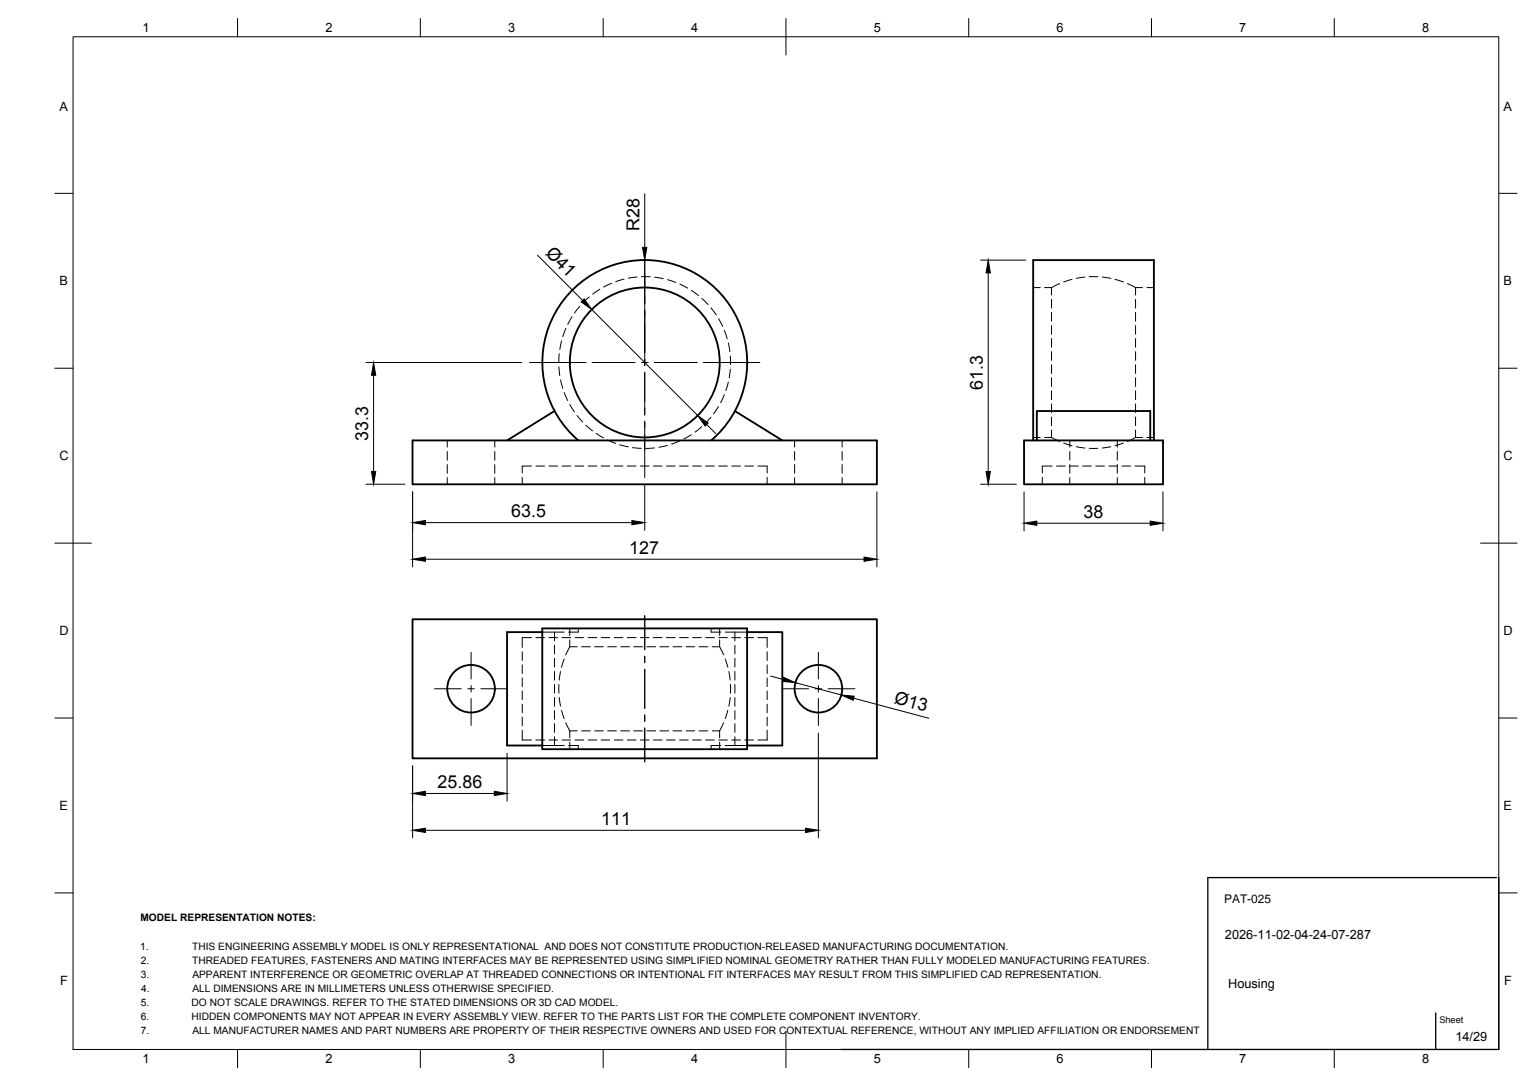
ISO-10303-21;
HEADER;
/* Generated by software containing ST-Developer
 * from STEP Tools, Inc. (www.steptools.com) 
 */

FILE_DESCRIPTION(
/* description */ ('Counter shaft with two pulleys and keyed hub'),
/* implementation_level */ '2;1');

FILE_NAME(
/* name */ 'Housing.step',
/* time_stamp */ '2026-10-27T10:46:10-07:00',
/* author */ (''),
/* organization */ (''),
/* preprocessor_version */ 'ST-DEVELOPER v20.2',
/* originating_system */ 'Autodesk Translation Framework v15.17.0.0',
/* authorisation */ '');

FILE_SCHEMA (('AUTOMOTIVE_DESIGN { 1 0 10303 214 3 1 1 }'));
ENDSEC;

DATA;
#10=MECHANICAL_DESIGN_GEOMETRIC_PRESENTATION_REPRESENTATION('',(#297),#10821);
#238=SPHERICAL_SURFACE('',#5956,2.35);
#247=SHAPE_REPRESENTATION_RELATIONSHIP('SRR','None',#10934,#272);
#272=ADVANCED_BREP_SHAPE_REPRESENTATION('',(#323),#10802);
#297=STYLED_ITEM('',(#11114),#323);
#323=MANIFOLD_SOLID_BREP('Body1',#5580);
#356=FACE_BOUND('',#959,.T.);
#357=FACE_BOUND('',#960,.T.);
#358=FACE_BOUND('',#968,.T.);
#359=FACE_BOUND('',#969,.T.);
#360=FACE_BOUND('',#970,.T.);
#361=FACE_BOUND('',#973,.T.);
#362=FACE_BOUND('',#975,.T.);
#363=FACE_BOUND('',#988,.T.);
#364=FACE_BOUND('',#989,.T.);
#365=FACE_BOUND('',#990,.T.);
#457=PLANE('',#5958);
#458=PLANE('',#5960);
#459=PLANE('',#5962);
#460=PLANE('',#5964);
#461=PLANE('',#5965);
#462=PLANE('',#5967);
#463=PLANE('',#5968);
#464=PLANE('',#5974);
#465=PLANE('',#5975);
#466=PLANE('',#5976);
#467=PLANE('',#5977);
#468=PLANE('',#5978);
#469=PLANE('',#5979);
#470=PLANE('',#5980);
#471=PLANE('',#5985);
#472=PLANE('',#5986);
#473=PLANE('',#5987);
#474=PLANE('',#5988);
#475=PLANE('',#5989);
#626=FACE_OUTER_BOUND('',#956,.T.);
#627=FACE_OUTER_BOUND('',#957,.T.);
#628=FACE_OUTER_BOUND('',#958,.T.);
#629=FACE_OUTER_BOUND('',#961,.T.);
#630=FACE_OUTER_BOUND('',#962,.T.);
#631=FACE_OUTER_BOUND('',#963,.T.);
#632=FACE_OUTER_BOUND('',#964,.T.);
#633=FACE_OUTER_BOUND('',#965,.T.);
#634=FACE_OUTER_BOUND('',#966,.T.);
#635=FACE_OUTER_BOUND('',#967,.T.);
#636=FACE_OUTER_BOUND('',#971,.T.);
#637=FACE_OUTER_BOUND('',#972,.T.);
#638=FACE_OUTER_BOUND('',#974,.T.);
#639=FACE_OUTER_BOUND('',#976,.T.);
#640=FACE_OUTER_BOUND('',#977,.T.);
#641=FACE_OUTER_BOUND('',#978,.T.);
#642=FACE_OUTER_BOUND('',#979,.T.);
#643=FACE_OUTER_BOUND('',#980,.T.);
#644=FACE_OUTER_BOUND('',#981,.T.);
#645=FACE_OUTER_BOUND('',#982,.T.);
#646=FACE_OUTER_BOUND('',#983,.T.);
#647=FACE_OUTER_BOUND('',#984,.T.);
#648=FACE_OUTER_BOUND('',#985,.T.);
#649=FACE_OUTER_BOUND('',#986,.T.);
#650=FACE_OUTER_BOUND('',#987,.T.);
#956=EDGE_LOOP('',(#3773,#3774,#3775,#3776));
#957=EDGE_LOOP('',(#3777,#3778,#3779,#3780));
#958=EDGE_LOOP('',(#3781,#3782));
#959=EDGE_LOOP('',(#3783));
#960=EDGE_LOOP('',(#3784));
#961=EDGE_LOOP('',(#3785,#3786,#3787));
#962=EDGE_LOOP('',(#3788,#3789,#3790));
#963=EDGE_LOOP('',(#3791,#3792,#3793));
#964=EDGE_LOOP('',(#3794,#3795,#3796,#3797));
#965=EDGE_LOOP('',(#3798,#3799,#3800));
#966=EDGE_LOOP('',(#3801,#3802,#3803,#3804));
#967=EDGE_LOOP('',(#3805,#3806,#3807,#3808));
#968=EDGE_LOOP('',(#3809));
#969=EDGE_LOOP('',(#3810));
#970=EDGE_LOOP('',(#3811,#3812,#3813,#3814,#3815,#3816,#3817,#3818,#3819,
#3820,#3821,#3822));
#971=EDGE_LOOP('',(#3823,#3824,#3825,#3826,#3827,#3828,#3829,#3830,#3831,
#3832,#3833,#3834));
#972=EDGE_LOOP('',(#3835,#3836));
#973=EDGE_LOOP('',(#3837));
#974=EDGE_LOOP('',(#3838,#3839));
#975=EDGE_LOOP('',(#3840));
#976=EDGE_LOOP('',(#3841,#3842,#3843,#3844));
#977=EDGE_LOOP('',(#3845,#3846,#3847,#3848));
#978=EDGE_LOOP('',(#3849,#3850,#3851,#3852));
#979=EDGE_LOOP('',(#3853,#3854,#3855,#3856));
#980=EDGE_LOOP('',(#3857,#3858,#3859,#3860));
#981=EDGE_LOOP('',(#3861,#3862,#3863,#3864));
#982=EDGE_LOOP('',(#3865,#3866,#3867,#3868));
#983=EDGE_LOOP('',(#3869,#3870,#3871,#3872));
#984=EDGE_LOOP('',(#3873,#3874,#3875,#3876));
#985=EDGE_LOOP('',(#3877,#3878,#3879,#3880));
#986=EDGE_LOOP('',(#3881,#3882,#3883,#3884));
#987=EDGE_LOOP('',(#3885,#3886,#3887,#3888));
#988=EDGE_LOOP('',(#3889,#3890,#3891,#3892));
#989=EDGE_LOOP('',(#3893));
#990=EDGE_LOOP('',(#3894));
#1355=LINE('',#8485,#1744);
#1356=LINE('',#8491,#1745);
#1357=LINE('',#8500,#1746);
#1358=LINE('',#8502,#1747);
#1359=LINE('',#8507,#1748);
#1360=LINE('',#8510,#1749);
#1361=LINE('',#8514,#1750);
#1362=LINE('',#8517,#1751);
#1363=LINE('',#8519,#1752);
#1364=LINE('',#8520,#1753);
#1365=LINE('',#8524,#1754);
#1366=LINE('',#8526,#1755);
#1367=LINE('',#8529,#1756);
#1368=LINE('',#8530,#1757);
#1369=LINE('',#8534,#1758);
#1370=LINE('',#8536,#1759);
#1371=LINE('',#8538,#1760);
#1372=LINE('',#8539,#1761);
#1373=LINE('',#8545,#1762);
#1374=LINE('',#8547,#1763);
#1375=LINE('',#8548,#1764);
#1376=LINE('',#8550,#1765);
#1377=LINE('',#8552,#1766);
#1378=LINE('',#8553,#1767);
#1379=LINE('',#8562,#1768);
#1380=LINE('',#8564,#1769);
#1381=LINE('',#8566,#1770);
#1382=LINE('',#8567,#1771);
#1383=LINE('',#8570,#1772);
#1384=LINE('',#8572,#1773);
#1385=LINE('',#8573,#1774);
#1386=LINE('',#8576,#1775);
#1387=LINE('',#8578,#1776);
#1388=LINE('',#8579,#1777);
#1389=LINE('',#8581,#1778);
#1390=LINE('',#8582,#1779);
#1391=LINE('',#8587,#1780);
#1392=LINE('',#8591,#1781);
#1393=LINE('',#8595,#1782);
#1394=LINE('',#8596,#1783);
#1395=LINE('',#8597,#1784);
#1396=LINE('',#8600,#1785);
#1397=LINE('',#8601,#1786);
#1398=LINE('',#8604,#1787);
#1399=LINE('',#8605,#1788);
#1400=LINE('',#8607,#1789);
#1744=VECTOR('',#6757,2.05);
#1745=VECTOR('',#6764,2.05);
#1746=VECTOR('',#6773,1.);
#1747=VECTOR('',#6774,1.);
#1748=VECTOR('',#6779,1.);
#1749=VECTOR('',#6782,1.);
#1750=VECTOR('',#6785,1.);
#1751=VECTOR('',#6788,1.);
#1752=VECTOR('',#6791,1.);
#1753=VECTOR('',#6792,1.);
#1754=VECTOR('',#6795,1.);
#1755=VECTOR('',#6796,1.);
#1756=VECTOR('',#6801,1.);
#1757=VECTOR('',#6802,1.);
#1758=VECTOR('',#6805,1.);
#1759=VECTOR('',#6806,1.);
#1760=VECTOR('',#6807,1.);
#1761=VECTOR('',#6808,1.);
#1762=VECTOR('',#6813,1.);
#1763=VECTOR('',#6814,1.);
#1764=VECTOR('',#6815,1.);
#1765=VECTOR('',#6816,1.);
#1766=VECTOR('',#6817,1.);
#1767=VECTOR('',#6818,1.);
#1768=VECTOR('',#6831,1.);
#1769=VECTOR('',#6832,1.);
#1770=VECTOR('',#6833,1.);
#1771=VECTOR('',#6834,1.);
#1772=VECTOR('',#6837,1.);
#1773=VECTOR('',#6838,1.);
#1774=VECTOR('',#6839,1.);
#1775=VECTOR('',#6842,1.);
#1776=VECTOR('',#6843,1.);
#1777=VECTOR('',#6844,1.);
#1778=VECTOR('',#6847,1.);
#1779=VECTOR('',#6848,1.);
#1780=VECTOR('',#6855,0.65);
#1781=VECTOR('',#6860,0.65);
#1782=VECTOR('',#6863,1.);
#1783=VECTOR('',#6864,1.);
#1784=VECTOR('',#6865,1.);
#1785=VECTOR('',#6868,1.);
#1786=VECTOR('',#6869,1.);
#1787=VECTOR('',#6872,1.);
#1788=VECTOR('',#6873,1.);
#1789=VECTOR('',#6876,1.);
#2109=CIRCLE('',#5951,2.05);
#2110=CIRCLE('',#5952,2.05);
#2111=CIRCLE('',#5954,2.05);
#2112=CIRCLE('',#5955,2.05);
#2113=CIRCLE('',#5957,2.35);
#2114=CIRCLE('',#5959,2.8);
#2115=CIRCLE('',#5961,2.8);
#2116=CIRCLE('',#5963,2.8);
#2117=CIRCLE('',#5966,2.8);
#2118=CIRCLE('',#5969,0.65);
#2119=CIRCLE('',#5970,0.65);
#2120=CIRCLE('',#5972,2.8);
#2121=CIRCLE('',#5973,2.8);
#2122=CIRCLE('',#5982,0.65);
#2123=CIRCLE('',#5984,0.65);
#2432=VERTEX_POINT('',#8482);
#2433=VERTEX_POINT('',#8484);
#2434=VERTEX_POINT('',#8488);
#2435=VERTEX_POINT('',#8490);
#2436=VERTEX_POINT('',#8494);
#2437=VERTEX_POINT('',#8495);
#2438=VERTEX_POINT('',#8498);
#2439=VERTEX_POINT('',#8499);
#2440=VERTEX_POINT('',#8501);
#2441=VERTEX_POINT('',#8505);
#2442=VERTEX_POINT('',#8506);
#2443=VERTEX_POINT('',#8508);
#2444=VERTEX_POINT('',#8512);
#2445=VERTEX_POINT('',#8513);
#2446=VERTEX_POINT('',#8515);
#2447=VERTEX_POINT('',#8522);
#2448=VERTEX_POINT('',#8523);
#2449=VERTEX_POINT('',#8525);
#2450=VERTEX_POINT('',#8532);
#2451=VERTEX_POINT('',#8533);
#2452=VERTEX_POINT('',#8535);
#2453=VERTEX_POINT('',#8537);
#2454=VERTEX_POINT('',#8540);
#2455=VERTEX_POINT('',#8542);
#2456=VERTEX_POINT('',#8544);
#2457=VERTEX_POINT('',#8546);
#2458=VERTEX_POINT('',#8549);
#2459=VERTEX_POINT('',#8551);
#2460=VERTEX_POINT('',#8560);
#2461=VERTEX_POINT('',#8561);
#2462=VERTEX_POINT('',#8563);
#2463=VERTEX_POINT('',#8565);
#2464=VERTEX_POINT('',#8569);
#2465=VERTEX_POINT('',#8571);
#2466=VERTEX_POINT('',#8575);
#2467=VERTEX_POINT('',#8577);
#2468=VERTEX_POINT('',#8585);
#2469=VERTEX_POINT('',#8589);
#2470=VERTEX_POINT('',#8593);
#2471=VERTEX_POINT('',#8594);
#2472=VERTEX_POINT('',#8599);
#2473=VERTEX_POINT('',#8603);
#2959=EDGE_CURVE('',#2432,#2432,#2109,.T.);
#2960=EDGE_CURVE('',#2432,#2433,#1355,.T.);
#2961=EDGE_CURVE('',#2433,#2433,#2110,.T.);
#2962=EDGE_CURVE('',#2434,#2434,#2111,.T.);
#2963=EDGE_CURVE('',#2434,#2435,#1356,.T.);
#2964=EDGE_CURVE('',#2435,#2435,#2112,.T.);
#2965=EDGE_CURVE('',#2436,#2437,#2113,.T.);
#2966=EDGE_CURVE('',#2438,#2439,#1357,.T.);
#2967=EDGE_CURVE('',#2438,#2440,#1358,.T.);
#2968=EDGE_CURVE('',#2439,#2440,#2114,.T.);
#2969=EDGE_CURVE('',#2441,#2442,#1359,.T.);
#2970=EDGE_CURVE('',#2443,#2441,#2115,.T.);
#2971=EDGE_CURVE('',#2443,#2442,#1360,.T.);
#2972=EDGE_CURVE('',#2444,#2445,#1361,.T.);
#2973=EDGE_CURVE('',#2446,#2444,#2116,.T.);
#2974=EDGE_CURVE('',#2446,#2445,#1362,.T.);
#2975=EDGE_CURVE('',#2445,#2438,#1363,.T.);
#2976=EDGE_CURVE('',#2440,#2446,#1364,.T.);
#2977=EDGE_CURVE('',#2447,#2448,#1365,.T.);
#2978=EDGE_CURVE('',#2447,#2449,#1366,.T.);
#2979=EDGE_CURVE('',#2448,#2449,#2117,.T.);
#2980=EDGE_CURVE('',#2442,#2447,#1367,.T.);
#2981=EDGE_CURVE('',#2449,#2443,#1368,.T.);
#2982=EDGE_CURVE('',#2450,#2451,#1369,.T.);
#2983=EDGE_CURVE('',#2451,#2452,#1370,.T.);
#2984=EDGE_CURVE('',#2452,#2453,#1371,.T.);
#2985=EDGE_CURVE('',#2453,#2450,#1372,.T.);
#2986=EDGE_CURVE('',#2454,#2454,#2118,.T.);
#2987=EDGE_CURVE('',#2455,#2455,#2119,.T.);
#2988=EDGE_CURVE('',#2448,#2456,#1373,.T.);
#2989=EDGE_CURVE('',#2456,#2457,#1374,.T.);
#2990=EDGE_CURVE('',#2457,#2444,#1375,.T.);
#2991=EDGE_CURVE('',#2439,#2458,#1376,.T.);
#2992=EDGE_CURVE('',#2458,#2459,#1377,.T.);
#2993=EDGE_CURVE('',#2459,#2441,#1378,.T.);
#2994=EDGE_CURVE('',#2458,#2459,#2120,.T.);
#2995=EDGE_CURVE('',#2456,#2457,#2121,.T.);
#2996=EDGE_CURVE('',#2460,#2461,#1379,.T.);
#2997=EDGE_CURVE('',#2460,#2462,#1380,.T.);
#2998=EDGE_CURVE('',#2462,#2463,#1381,.T.);
#2999=EDGE_CURVE('',#2461,#2463,#1382,.T.);
#3000=EDGE_CURVE('',#2464,#2460,#1383,.T.);
#3001=EDGE_CURVE('',#2464,#2465,#1384,.T.);
#3002=EDGE_CURVE('',#2465,#2462,#1385,.T.);
#3003=EDGE_CURVE('',#2466,#2464,#1386,.T.);
#3004=EDGE_CURVE('',#2466,#2467,#1387,.T.);
#3005=EDGE_CURVE('',#2467,#2465,#1388,.T.);
#3006=EDGE_CURVE('',#2461,#2466,#1389,.T.);
#3007=EDGE_CURVE('',#2463,#2467,#1390,.T.);
#3008=EDGE_CURVE('',#2468,#2468,#2122,.T.);
#3009=EDGE_CURVE('',#2468,#2455,#1391,.T.);
#3010=EDGE_CURVE('',#2469,#2469,#2123,.T.);
#3011=EDGE_CURVE('',#2469,#2454,#1392,.T.);
#3012=EDGE_CURVE('',#2470,#2471,#1393,.T.);
#3013=EDGE_CURVE('',#2471,#2450,#1394,.T.);
#3014=EDGE_CURVE('',#2470,#2453,#1395,.T.);
#3015=EDGE_CURVE('',#2472,#2470,#1396,.T.);
#3016=EDGE_CURVE('',#2472,#2452,#1397,.T.);
#3017=EDGE_CURVE('',#2473,#2472,#1398,.T.);
#3018=EDGE_CURVE('',#2473,#2451,#1399,.T.);
#3019=EDGE_CURVE('',#2471,#2473,#1400,.T.);
#3773=ORIENTED_EDGE('',*,*,#2959,.F.);
#3774=ORIENTED_EDGE('',*,*,#2960,.T.);
#3775=ORIENTED_EDGE('',*,*,#2961,.F.);
#3776=ORIENTED_EDGE('',*,*,#2960,.F.);
#3777=ORIENTED_EDGE('',*,*,#2962,.F.);
#3778=ORIENTED_EDGE('',*,*,#2963,.T.);
#3779=ORIENTED_EDGE('',*,*,#2964,.F.);
#3780=ORIENTED_EDGE('',*,*,#2963,.F.);
#3781=ORIENTED_EDGE('',*,*,#2965,.T.);
#3782=ORIENTED_EDGE('',*,*,#2965,.F.);
#3783=ORIENTED_EDGE('',*,*,#2962,.T.);
#3784=ORIENTED_EDGE('',*,*,#2961,.T.);
#3785=ORIENTED_EDGE('',*,*,#2966,.F.);
#3786=ORIENTED_EDGE('',*,*,#2967,.T.);
#3787=ORIENTED_EDGE('',*,*,#2968,.F.);
#3788=ORIENTED_EDGE('',*,*,#2969,.F.);
#3789=ORIENTED_EDGE('',*,*,#2970,.F.);
#3790=ORIENTED_EDGE('',*,*,#2971,.T.);
#3791=ORIENTED_EDGE('',*,*,#2972,.F.);
#3792=ORIENTED_EDGE('',*,*,#2973,.F.);
#3793=ORIENTED_EDGE('',*,*,#2974,.T.);
#3794=ORIENTED_EDGE('',*,*,#2975,.F.);
#3795=ORIENTED_EDGE('',*,*,#2974,.F.);
#3796=ORIENTED_EDGE('',*,*,#2976,.F.);
#3797=ORIENTED_EDGE('',*,*,#2967,.F.);
#3798=ORIENTED_EDGE('',*,*,#2977,.F.);
#3799=ORIENTED_EDGE('',*,*,#2978,.T.);
#3800=ORIENTED_EDGE('',*,*,#2979,.F.);
#3801=ORIENTED_EDGE('',*,*,#2980,.F.);
#3802=ORIENTED_EDGE('',*,*,#2971,.F.);
#3803=ORIENTED_EDGE('',*,*,#2981,.F.);
#3804=ORIENTED_EDGE('',*,*,#2978,.F.);
#3805=ORIENTED_EDGE('',*,*,#2982,.T.);
#3806=ORIENTED_EDGE('',*,*,#2983,.T.);
#3807=ORIENTED_EDGE('',*,*,#2984,.T.);
#3808=ORIENTED_EDGE('',*,*,#2985,.T.);
#3809=ORIENTED_EDGE('',*,*,#2986,.T.);
#3810=ORIENTED_EDGE('',*,*,#2987,.T.);
#3811=ORIENTED_EDGE('',*,*,#2969,.T.);
#3812=ORIENTED_EDGE('',*,*,#2980,.T.);
#3813=ORIENTED_EDGE('',*,*,#2977,.T.);
#3814=ORIENTED_EDGE('',*,*,#2988,.T.);
#3815=ORIENTED_EDGE('',*,*,#2989,.T.);
#3816=ORIENTED_EDGE('',*,*,#2990,.T.);
#3817=ORIENTED_EDGE('',*,*,#2972,.T.);
#3818=ORIENTED_EDGE('',*,*,#2975,.T.);
#3819=ORIENTED_EDGE('',*,*,#2966,.T.);
#3820=ORIENTED_EDGE('',*,*,#2991,.T.);
#3821=ORIENTED_EDGE('',*,*,#2992,.T.);
#3822=ORIENTED_EDGE('',*,*,#2993,.T.);
#3823=ORIENTED_EDGE('',*,*,#2970,.T.);
#3824=ORIENTED_EDGE('',*,*,#2993,.F.);
#3825=ORIENTED_EDGE('',*,*,#2994,.F.);
#3826=ORIENTED_EDGE('',*,*,#2991,.F.);
#3827=ORIENTED_EDGE('',*,*,#2968,.T.);
#3828=ORIENTED_EDGE('',*,*,#2976,.T.);
#3829=ORIENTED_EDGE('',*,*,#2973,.T.);
#3830=ORIENTED_EDGE('',*,*,#2990,.F.);
#3831=ORIENTED_EDGE('',*,*,#2995,.F.);
#3832=ORIENTED_EDGE('',*,*,#2988,.F.);
#3833=ORIENTED_EDGE('',*,*,#2979,.T.);
#3834=ORIENTED_EDGE('',*,*,#2981,.T.);
#3835=ORIENTED_EDGE('',*,*,#2989,.F.);
#3836=ORIENTED_EDGE('',*,*,#2995,.T.);
#3837=ORIENTED_EDGE('',*,*,#2959,.T.);
#3838=ORIENTED_EDGE('',*,*,#2992,.F.);
#3839=ORIENTED_EDGE('',*,*,#2994,.T.);
#3840=ORIENTED_EDGE('',*,*,#2964,.T.);
#3841=ORIENTED_EDGE('',*,*,#2996,.F.);
#3842=ORIENTED_EDGE('',*,*,#2997,.T.);
#3843=ORIENTED_EDGE('',*,*,#2998,.T.);
#3844=ORIENTED_EDGE('',*,*,#2999,.F.);
#3845=ORIENTED_EDGE('',*,*,#3000,.F.);
#3846=ORIENTED_EDGE('',*,*,#3001,.T.);
#3847=ORIENTED_EDGE('',*,*,#3002,.T.);
#3848=ORIENTED_EDGE('',*,*,#2997,.F.);
#3849=ORIENTED_EDGE('',*,*,#3003,.F.);
#3850=ORIENTED_EDGE('',*,*,#3004,.T.);
#3851=ORIENTED_EDGE('',*,*,#3005,.T.);
#3852=ORIENTED_EDGE('',*,*,#3001,.F.);
#3853=ORIENTED_EDGE('',*,*,#3006,.F.);
#3854=ORIENTED_EDGE('',*,*,#2999,.T.);
#3855=ORIENTED_EDGE('',*,*,#3007,.T.);
#3856=ORIENTED_EDGE('',*,*,#3004,.F.);
#3857=ORIENTED_EDGE('',*,*,#3007,.F.);
#3858=ORIENTED_EDGE('',*,*,#2998,.F.);
#3859=ORIENTED_EDGE('',*,*,#3002,.F.);
#3860=ORIENTED_EDGE('',*,*,#3005,.F.);
#3861=ORIENTED_EDGE('',*,*,#3008,.F.);
#3862=ORIENTED_EDGE('',*,*,#3009,.T.);
#3863=ORIENTED_EDGE('',*,*,#2987,.F.);
#3864=ORIENTED_EDGE('',*,*,#3009,.F.);
#3865=ORIENTED_EDGE('',*,*,#3010,.F.);
#3866=ORIENTED_EDGE('',*,*,#3011,.T.);
#3867=ORIENTED_EDGE('',*,*,#2986,.F.);
#3868=ORIENTED_EDGE('',*,*,#3011,.F.);
#3869=ORIENTED_EDGE('',*,*,#3012,.T.);
#3870=ORIENTED_EDGE('',*,*,#3013,.T.);
#3871=ORIENTED_EDGE('',*,*,#2985,.F.);
#3872=ORIENTED_EDGE('',*,*,#3014,.F.);
#3873=ORIENTED_EDGE('',*,*,#3015,.T.);
#3874=ORIENTED_EDGE('',*,*,#3014,.T.);
#3875=ORIENTED_EDGE('',*,*,#2984,.F.);
#3876=ORIENTED_EDGE('',*,*,#3016,.F.);
#3877=ORIENTED_EDGE('',*,*,#3017,.T.);
#3878=ORIENTED_EDGE('',*,*,#3016,.T.);
#3879=ORIENTED_EDGE('',*,*,#2983,.F.);
#3880=ORIENTED_EDGE('',*,*,#3018,.F.);
#3881=ORIENTED_EDGE('',*,*,#3019,.T.);
#3882=ORIENTED_EDGE('',*,*,#3018,.T.);
#3883=ORIENTED_EDGE('',*,*,#2982,.F.);
#3884=ORIENTED_EDGE('',*,*,#3013,.F.);
#3885=ORIENTED_EDGE('',*,*,#3019,.F.);
#3886=ORIENTED_EDGE('',*,*,#3012,.F.);
#3887=ORIENTED_EDGE('',*,*,#3015,.F.);
#3888=ORIENTED_EDGE('',*,*,#3017,.F.);
#3889=ORIENTED_EDGE('',*,*,#2996,.T.);
#3890=ORIENTED_EDGE('',*,*,#3006,.T.);
#3891=ORIENTED_EDGE('',*,*,#3003,.T.);
#3892=ORIENTED_EDGE('',*,*,#3000,.T.);
#3893=ORIENTED_EDGE('',*,*,#3008,.T.);
#3894=ORIENTED_EDGE('',*,*,#3010,.T.);
#5125=CYLINDRICAL_SURFACE('',#5950,2.05);
#5126=CYLINDRICAL_SURFACE('',#5953,2.05);
#5127=CYLINDRICAL_SURFACE('',#5971,2.8);
#5128=CYLINDRICAL_SURFACE('',#5981,0.65);
#5129=CYLINDRICAL_SURFACE('',#5983,0.65);
#5297=ADVANCED_FACE('',(#626),#5125,.F.);
#5298=ADVANCED_FACE('',(#627),#5126,.F.);
#5299=ADVANCED_FACE('',(#628,#356,#357),#238,.F.);
#5300=ADVANCED_FACE('',(#629),#457,.T.);
#5301=ADVANCED_FACE('',(#630),#458,.T.);
#5302=ADVANCED_FACE('',(#631),#459,.T.);
#5303=ADVANCED_FACE('',(#632),#460,.T.);
#5304=ADVANCED_FACE('',(#633),#461,.T.);
#5305=ADVANCED_FACE('',(#634),#462,.T.);
#5306=ADVANCED_FACE('',(#635,#358,#359,#360),#463,.T.);
#5307=ADVANCED_FACE('',(#636),#5127,.T.);
#5308=ADVANCED_FACE('',(#637,#361),#464,.F.);
#5309=ADVANCED_FACE('',(#638,#362),#465,.T.);
#5310=ADVANCED_FACE('',(#639),#466,.F.);
#5311=ADVANCED_FACE('',(#640),#467,.F.);
#5312=ADVANCED_FACE('',(#641),#468,.F.);
#5313=ADVANCED_FACE('',(#642),#469,.F.);
#5314=ADVANCED_FACE('',(#643),#470,.F.);
#5315=ADVANCED_FACE('',(#644),#5128,.F.);
#5316=ADVANCED_FACE('',(#645),#5129,.F.);
#5317=ADVANCED_FACE('',(#646),#471,.T.);
#5318=ADVANCED_FACE('',(#647),#472,.T.);
#5319=ADVANCED_FACE('',(#648),#473,.T.);
#5320=ADVANCED_FACE('',(#649),#474,.T.);
#5321=ADVANCED_FACE('',(#650,#363,#364,#365),#475,.F.);
#5580=CLOSED_SHELL('',(#5297,#5298,#5299,#5300,#5301,#5302,#5303,#5304,
#5305,#5306,#5307,#5308,#5309,#5310,#5311,#5312,#5313,#5314,#5315,#5316,
#5317,#5318,#5319,#5320,#5321));
#5949=AXIS2_PLACEMENT_3D('',#8480,#6751,#6752);
#5950=AXIS2_PLACEMENT_3D('',#8481,#6753,#6754);
#5951=AXIS2_PLACEMENT_3D('',#8483,#6755,#6756);
#5952=AXIS2_PLACEMENT_3D('',#8486,#6758,#6759);
#5953=AXIS2_PLACEMENT_3D('',#8487,#6760,#6761);
#5954=AXIS2_PLACEMENT_3D('',#8489,#6762,#6763);
#5955=AXIS2_PLACEMENT_3D('',#8492,#6765,#6766);
#5956=AXIS2_PLACEMENT_3D('',#8493,#6767,#6768);
#5957=AXIS2_PLACEMENT_3D('',#8496,#6769,#6770);
#5958=AXIS2_PLACEMENT_3D('',#8497,#6771,#6772);
#5959=AXIS2_PLACEMENT_3D('',#8503,#6775,#6776);
#5960=AXIS2_PLACEMENT_3D('',#8504,#6777,#6778);
#5961=AXIS2_PLACEMENT_3D('',#8509,#6780,#6781);
#5962=AXIS2_PLACEMENT_3D('',#8511,#6783,#6784);
#5963=AXIS2_PLACEMENT_3D('',#8516,#6786,#6787);
#5964=AXIS2_PLACEMENT_3D('',#8518,#6789,#6790);
#5965=AXIS2_PLACEMENT_3D('',#8521,#6793,#6794);
#5966=AXIS2_PLACEMENT_3D('',#8527,#6797,#6798);
#5967=AXIS2_PLACEMENT_3D('',#8528,#6799,#6800);
#5968=AXIS2_PLACEMENT_3D('',#8531,#6803,#6804);
#5969=AXIS2_PLACEMENT_3D('',#8541,#6809,#6810);
#5970=AXIS2_PLACEMENT_3D('',#8543,#6811,#6812);
#5971=AXIS2_PLACEMENT_3D('',#8554,#6819,#6820);
#5972=AXIS2_PLACEMENT_3D('',#8555,#6821,#6822);
#5973=AXIS2_PLACEMENT_3D('',#8556,#6823,#6824);
#5974=AXIS2_PLACEMENT_3D('',#8557,#6825,#6826);
#5975=AXIS2_PLACEMENT_3D('',#8558,#6827,#6828);
#5976=AXIS2_PLACEMENT_3D('',#8559,#6829,#6830);
#5977=AXIS2_PLACEMENT_3D('',#8568,#6835,#6836);
#5978=AXIS2_PLACEMENT_3D('',#8574,#6840,#6841);
#5979=AXIS2_PLACEMENT_3D('',#8580,#6845,#6846);
#5980=AXIS2_PLACEMENT_3D('',#8583,#6849,#6850);
#5981=AXIS2_PLACEMENT_3D('',#8584,#6851,#6852);
#5982=AXIS2_PLACEMENT_3D('',#8586,#6853,#6854);
#5983=AXIS2_PLACEMENT_3D('',#8588,#6856,#6857);
#5984=AXIS2_PLACEMENT_3D('',#8590,#6858,#6859);
#5985=AXIS2_PLACEMENT_3D('',#8592,#6861,#6862);
#5986=AXIS2_PLACEMENT_3D('',#8598,#6866,#6867);
#5987=AXIS2_PLACEMENT_3D('',#8602,#6870,#6871);
#5988=AXIS2_PLACEMENT_3D('',#8606,#6874,#6875);
#5989=AXIS2_PLACEMENT_3D('',#8608,#6877,#6878);
#6751=DIRECTION('axis',(0.,0.,1.));
#6752=DIRECTION('refdir',(1.,0.,0.));
#6753=DIRECTION('center_axis',(0.,1.,0.));
#6754=DIRECTION('ref_axis',(1.,0.,0.));
#6755=DIRECTION('center_axis',(0.,1.,0.));
#6756=DIRECTION('ref_axis',(1.,0.,0.));
#6757=DIRECTION('',(0.,1.,0.));
#6758=DIRECTION('center_axis',(0.,-1.,0.));
#6759=DIRECTION('ref_axis',(1.,0.,0.));
#6760=DIRECTION('center_axis',(0.,1.,0.));
#6761=DIRECTION('ref_axis',(1.,0.,0.));
#6762=DIRECTION('center_axis',(0.,1.,0.));
#6763=DIRECTION('ref_axis',(1.,0.,0.));
#6764=DIRECTION('',(0.,1.,0.));
#6765=DIRECTION('center_axis',(0.,-1.,0.));
#6766=DIRECTION('ref_axis',(1.,0.,0.));
#6767=DIRECTION('center_axis',(6.12323399573677E-17,0.,1.));
#6768=DIRECTION('ref_axis',(1.,0.,0.));
#6769=DIRECTION('center_axis',(-1.22464679914735E-16,1.,0.));
#6770=DIRECTION('ref_axis',(-1.,-1.22464679914735E-16,0.));
#6771=DIRECTION('center_axis',(0.,1.,0.));
#6772=DIRECTION('ref_axis',(0.,0.,1.));
#6773=DIRECTION('',(1.,0.,0.));
#6774=DIRECTION('',(0.850265146687862,0.,0.526354614616295));
#6775=DIRECTION('center_axis',(0.,1.,0.));
#6776=DIRECTION('ref_axis',(1.,0.,0.));
#6777=DIRECTION('center_axis',(0.,1.,0.));
#6778=DIRECTION('ref_axis',(0.,0.,1.));
#6779=DIRECTION('',(1.,0.,0.));
#6780=DIRECTION('center_axis',(0.,1.,0.));
#6781=DIRECTION('ref_axis',(1.,0.,0.));
#6782=DIRECTION('',(0.850265146687862,0.,-0.526354614616295));
#6783=DIRECTION('center_axis',(0.,-1.,0.));
#6784=DIRECTION('ref_axis',(0.,0.,-1.));
#6785=DIRECTION('',(-1.,0.,0.));
#6786=DIRECTION('center_axis',(0.,-1.,0.));
#6787=DIRECTION('ref_axis',(1.,0.,0.));
#6788=DIRECTION('',(-0.850265146687862,0.,-0.526354614616295));
#6789=DIRECTION('center_axis',(-0.526354614616295,0.,0.850265146687862));
#6790=DIRECTION('ref_axis',(0.850265146687862,0.,0.526354614616295));
#6791=DIRECTION('',(0.,1.,0.));
#6792=DIRECTION('',(0.,-1.,0.));
#6793=DIRECTION('center_axis',(0.,-1.,0.));
#6794=DIRECTION('ref_axis',(0.,0.,-1.));
#6795=DIRECTION('',(-1.,0.,0.));
#6796=DIRECTION('',(-0.850265146687862,0.,0.526354614616295));
#6797=DIRECTION('center_axis',(0.,-1.,0.));
#6798=DIRECTION('ref_axis',(1.,0.,0.));
#6799=DIRECTION('center_axis',(0.526354614616295,0.,0.850265146687862));
#6800=DIRECTION('ref_axis',(0.850265146687862,0.,-0.526354614616295));
#6801=DIRECTION('',(0.,-1.,0.));
#6802=DIRECTION('',(0.,1.,0.));
#6803=DIRECTION('center_axis',(0.,0.,1.));
#6804=DIRECTION('ref_axis',(1.,0.,0.));
#6805=DIRECTION('',(0.,-1.,0.));
#6806=DIRECTION('',(1.,0.,0.));
#6807=DIRECTION('',(0.,1.,0.));
#6808=DIRECTION('',(-1.,0.,0.));
#6809=DIRECTION('center_axis',(0.,0.,-1.));
#6810=DIRECTION('ref_axis',(1.,0.,0.));
#6811=DIRECTION('center_axis',(0.,0.,-1.));
#6812=DIRECTION('ref_axis',(1.,0.,0.));
#6813=DIRECTION('',(0.,-1.,0.));
#6814=DIRECTION('',(-1.,0.,0.));
#6815=DIRECTION('',(0.,1.,0.));
#6816=DIRECTION('',(0.,1.,0.));
#6817=DIRECTION('',(1.,0.,0.));
#6818=DIRECTION('',(0.,-1.,0.));
#6819=DIRECTION('center_axis',(0.,1.,0.));
#6820=DIRECTION('ref_axis',(6.12323399573677E-17,0.,1.));
#6821=DIRECTION('center_axis',(0.,1.,0.));
#6822=DIRECTION('ref_axis',(1.,0.,0.));
#6823=DIRECTION('center_axis',(0.,-1.,0.));
#6824=DIRECTION('ref_axis',(1.,0.,0.));
#6825=DIRECTION('center_axis',(0.,1.,0.));
#6826=DIRECTION('ref_axis',(1.,0.,0.));
#6827=DIRECTION('center_axis',(0.,1.,0.));
#6828=DIRECTION('ref_axis',(1.,0.,0.));
#6829=DIRECTION('center_axis',(0.,1.,0.));
#6830=DIRECTION('ref_axis',(-1.,0.,0.));
#6831=DIRECTION('',(-1.,0.,0.));
#6832=DIRECTION('',(0.,0.,1.));
#6833=DIRECTION('',(-1.,0.,0.));
#6834=DIRECTION('',(0.,0.,1.));
#6835=DIRECTION('center_axis',(1.,0.,0.));
#6836=DIRECTION('ref_axis',(0.,1.,0.));
#6837=DIRECTION('',(0.,1.,0.));
#6838=DIRECTION('',(0.,0.,1.));
#6839=DIRECTION('',(0.,1.,0.));
#6840=DIRECTION('center_axis',(0.,-1.,0.));
#6841=DIRECTION('ref_axis',(1.,0.,0.));
#6842=DIRECTION('',(1.,0.,0.));
#6843=DIRECTION('',(0.,0.,1.));
#6844=DIRECTION('',(1.,0.,0.));
#6845=DIRECTION('center_axis',(-1.,0.,0.));
#6846=DIRECTION('ref_axis',(0.,-1.,0.));
#6847=DIRECTION('',(0.,-1.,0.));
#6848=DIRECTION('',(0.,-1.,0.));
#6849=DIRECTION('center_axis',(0.,0.,1.));
#6850=DIRECTION('ref_axis',(1.,0.,0.));
#6851=DIRECTION('center_axis',(0.,0.,1.));
#6852=DIRECTION('ref_axis',(1.,0.,0.));
#6853=DIRECTION('center_axis',(0.,0.,1.));
#6854=DIRECTION('ref_axis',(1.,0.,0.));
#6855=DIRECTION('',(0.,0.,1.));
#6856=DIRECTION('center_axis',(0.,0.,1.));
#6857=DIRECTION('ref_axis',(1.,0.,0.));
#6858=DIRECTION('center_axis',(0.,0.,1.));
#6859=DIRECTION('ref_axis',(1.,0.,0.));
#6860=DIRECTION('',(0.,0.,1.));
#6861=DIRECTION('center_axis',(0.,1.,0.));
#6862=DIRECTION('ref_axis',(-1.,0.,0.));
#6863=DIRECTION('',(-1.,0.,0.));
#6864=DIRECTION('',(0.,0.,1.));
#6865=DIRECTION('',(0.,0.,1.));
#6866=DIRECTION('center_axis',(1.,0.,0.));
#6867=DIRECTION('ref_axis',(0.,1.,0.));
#6868=DIRECTION('',(0.,1.,0.));
#6869=DIRECTION('',(0.,0.,1.));
#6870=DIRECTION('center_axis',(0.,-1.,0.));
#6871=DIRECTION('ref_axis',(1.,0.,0.));
#6872=DIRECTION('',(1.,0.,0.));
#6873=DIRECTION('',(0.,0.,1.));
#6874=DIRECTION('center_axis',(-1.,0.,0.));
#6875=DIRECTION('ref_axis',(0.,-1.,0.));
#6876=DIRECTION('',(0.,-1.,0.));
#6877=DIRECTION('center_axis',(0.,0.,1.));
#6878=DIRECTION('ref_axis',(1.,0.,0.));
#8480=CARTESIAN_POINT('',(0.,0.,0.));
#8481=CARTESIAN_POINT('Origin',(0.,0.,0.));
#8482=CARTESIAN_POINT('',(-2.05,-1.65,2.51052593825207E-16));
#8483=CARTESIAN_POINT('Origin',(0.,-1.65,0.));
#8484=CARTESIAN_POINT('',(-2.05,-1.14891252930761,-2.51052593825207E-16));
#8485=CARTESIAN_POINT('',(-2.05,0.,2.51052593825207E-16));
#8486=CARTESIAN_POINT('Origin',(0.,-1.14891252930761,0.));
#8487=CARTESIAN_POINT('Origin',(0.,0.,0.));
#8488=CARTESIAN_POINT('',(-2.05,1.14891252930761,2.51052593825207E-16));
#8489=CARTESIAN_POINT('Origin',(0.,1.14891252930761,0.));
#8490=CARTESIAN_POINT('',(-2.05,1.65,-2.51052593825207E-16));
#8491=CARTESIAN_POINT('',(-2.05,0.,2.51052593825207E-16));
#8492=CARTESIAN_POINT('Origin',(0.,1.65,0.));
#8493=CARTESIAN_POINT('Origin',(0.,0.,0.));
#8494=CARTESIAN_POINT('',(-1.43895998899814E-16,-1.76221774462768E-32,-2.35));
#8495=CARTESIAN_POINT('',(-1.43895998899814E-16,-1.76221774462768E-32,2.35));
#8496=CARTESIAN_POINT('Origin',(0.,0.,0.));
#8497=CARTESIAN_POINT('Origin',(0.,1.55,-1.49));
#8498=CARTESIAN_POINT('',(-3.76384615384615,1.55,-2.13));
#8499=CARTESIAN_POINT('',(-1.81744325908679,1.55,-2.13));
#8500=CARTESIAN_POINT('',(0.,1.55,-2.13));
#8501=CARTESIAN_POINT('',(-2.46585583768694,1.55,-1.32648218523477));
#8502=CARTESIAN_POINT('',(-1.68,1.55,-0.84));
#8503=CARTESIAN_POINT('Origin',(0.,1.55,0.));
#8504=CARTESIAN_POINT('Origin',(0.,1.55,-1.49));
#8505=CARTESIAN_POINT('',(1.81744325908679,1.55,-2.13));
#8506=CARTESIAN_POINT('',(3.76384615384615,1.55,-2.13));
#8507=CARTESIAN_POINT('',(0.,1.55,-2.13));
#8508=CARTESIAN_POINT('',(2.46585583768694,1.55,-1.32648218523477));
#8509=CARTESIAN_POINT('Origin',(0.,1.55,0.));
#8510=CARTESIAN_POINT('',(3.78,1.55,-2.14));
#8511=CARTESIAN_POINT('Origin',(0.,-1.55,-1.49));
#8512=CARTESIAN_POINT('',(-1.81744325908679,-1.55,-2.13));
#8513=CARTESIAN_POINT('',(-3.76384615384615,-1.55,-2.13));
#8514=CARTESIAN_POINT('',(0.,-1.55,-2.13));
#8515=CARTESIAN_POINT('',(-2.46585583768694,-1.55,-1.32648218523477));
#8516=CARTESIAN_POINT('Origin',(0.,-1.55,0.));
#8517=CARTESIAN_POINT('',(-1.68,-1.55,-0.84));
#8518=CARTESIAN_POINT('Origin',(-3.78,0.,-2.14));
#8519=CARTESIAN_POINT('',(-3.76384615384615,0.,-2.13));
#8520=CARTESIAN_POINT('',(-2.46585583768694,0.,-1.32648218523477));
#8521=CARTESIAN_POINT('Origin',(0.,-1.55,-1.49));
#8522=CARTESIAN_POINT('',(3.76384615384615,-1.55,-2.13));
#8523=CARTESIAN_POINT('',(1.81744325908679,-1.55,-2.13));
#8524=CARTESIAN_POINT('',(0.,-1.55,-2.13));
#8525=CARTESIAN_POINT('',(2.46585583768694,-1.55,-1.32648218523477));
#8526=CARTESIAN_POINT('',(3.78,-1.55,-2.14));
#8527=CARTESIAN_POINT('Origin',(0.,-1.55,0.));
#8528=CARTESIAN_POINT('Origin',(1.68,0.,-0.84));
#8529=CARTESIAN_POINT('',(3.76384615384615,0.,-2.13));
#8530=CARTESIAN_POINT('',(2.46585583768694,0.,-1.32648218523477));
#8531=CARTESIAN_POINT('Origin',(0.,0.,-2.13));
#8532=CARTESIAN_POINT('',(-6.35,1.9,-2.13));
#8533=CARTESIAN_POINT('',(-6.35,-1.9,-2.13));
#8534=CARTESIAN_POINT('',(-6.35,1.9,-2.13));
#8535=CARTESIAN_POINT('',(6.35,-1.9,-2.13));
#8536=CARTESIAN_POINT('',(-6.35,-1.9,-2.13));
#8537=CARTESIAN_POINT('',(6.35,1.9,-2.13));
#8538=CARTESIAN_POINT('',(6.35,-1.9,-2.13));
#8539=CARTESIAN_POINT('',(6.35,1.9,-2.13));
#8540=CARTESIAN_POINT('',(4.1,7.9602041944578E-17,-2.13));
#8541=CARTESIAN_POINT('Origin',(4.75,0.,-2.13));
#8542=CARTESIAN_POINT('',(-5.4,7.9602041944578E-17,-2.13));
#8543=CARTESIAN_POINT('Origin',(-4.75,0.,-2.13));
#8544=CARTESIAN_POINT('',(1.81744325908679,-1.65,-2.13));
#8545=CARTESIAN_POINT('',(1.81744325908679,0.,-2.13));
#8546=CARTESIAN_POINT('',(-1.81744325908679,-1.65,-2.13));
#8547=CARTESIAN_POINT('',(0.,-1.65,-2.13));
#8548=CARTESIAN_POINT('',(-1.81744325908679,0.,-2.13));
#8549=CARTESIAN_POINT('',(-1.81744325908679,1.65,-2.13));
#8550=CARTESIAN_POINT('',(-1.81744325908679,0.,-2.13));
#8551=CARTESIAN_POINT('',(1.81744325908679,1.65,-2.13));
#8552=CARTESIAN_POINT('',(0.,1.65,-2.13));
#8553=CARTESIAN_POINT('',(1.81744325908679,0.,-2.13));
#8554=CARTESIAN_POINT('Origin',(0.,0.,0.));
#8555=CARTESIAN_POINT('Origin',(0.,1.65,0.));
#8556=CARTESIAN_POINT('Origin',(0.,-1.65,0.));
#8557=CARTESIAN_POINT('Origin',(0.,-1.65,0.));
#8558=CARTESIAN_POINT('Origin',(0.,1.65,0.));
#8559=CARTESIAN_POINT('Origin',(3.35,1.4,-3.33));
#8560=CARTESIAN_POINT('',(3.35,1.4,-3.33));
#8561=CARTESIAN_POINT('',(-3.35,1.4,-3.33));
#8562=CARTESIAN_POINT('',(1.675,1.4,-3.33));
#8563=CARTESIAN_POINT('',(3.35,1.4,-2.83));
#8564=CARTESIAN_POINT('',(3.35,1.4,-3.33));
#8565=CARTESIAN_POINT('',(-3.35,1.4,-2.83));
#8566=CARTESIAN_POINT('',(3.35,1.4,-2.83));
#8567=CARTESIAN_POINT('',(-3.35,1.4,-3.33));
#8568=CARTESIAN_POINT('Origin',(3.35,-1.4,-3.33));
#8569=CARTESIAN_POINT('',(3.35,-1.4,-3.33));
#8570=CARTESIAN_POINT('',(3.35,-0.7,-3.33));
#8571=CARTESIAN_POINT('',(3.35,-1.4,-2.83));
#8572=CARTESIAN_POINT('',(3.35,-1.4,-3.33));
#8573=CARTESIAN_POINT('',(3.35,-1.4,-2.83));
#8574=CARTESIAN_POINT('Origin',(-3.35,-1.4,-3.33));
#8575=CARTESIAN_POINT('',(-3.35,-1.4,-3.33));
#8576=CARTESIAN_POINT('',(-1.675,-1.4,-3.33));
#8577=CARTESIAN_POINT('',(-3.35,-1.4,-2.83));
#8578=CARTESIAN_POINT('',(-3.35,-1.4,-3.33));
#8579=CARTESIAN_POINT('',(-3.35,-1.4,-2.83));
#8580=CARTESIAN_POINT('Origin',(-3.35,1.4,-3.33));
#8581=CARTESIAN_POINT('',(-3.35,0.7,-3.33));
#8582=CARTESIAN_POINT('',(-3.35,1.4,-2.83));
#8583=CARTESIAN_POINT('Origin',(0.,0.,-2.83));
#8584=CARTESIAN_POINT('Origin',(-4.75,0.,-3.33));
#8585=CARTESIAN_POINT('',(-5.4,-7.9602041944578E-17,-3.33));
#8586=CARTESIAN_POINT('Origin',(-4.75,0.,-3.33));
#8587=CARTESIAN_POINT('',(-5.4,-7.9602041944578E-17,-3.33));
#8588=CARTESIAN_POINT('Origin',(4.75,0.,-3.33));
#8589=CARTESIAN_POINT('',(4.1,-7.9602041944578E-17,-3.33));
#8590=CARTESIAN_POINT('Origin',(4.75,0.,-3.33));
#8591=CARTESIAN_POINT('',(4.1,-7.9602041944578E-17,-3.33));
#8592=CARTESIAN_POINT('Origin',(6.35,1.9,-3.33));
#8593=CARTESIAN_POINT('',(6.35,1.9,-3.33));
#8594=CARTESIAN_POINT('',(-6.35,1.9,-3.33));
#8595=CARTESIAN_POINT('',(6.35,1.9,-3.33));
#8596=CARTESIAN_POINT('',(-6.35,1.9,-3.33));
#8597=CARTESIAN_POINT('',(6.35,1.9,-3.33));
#8598=CARTESIAN_POINT('Origin',(6.35,-1.9,-3.33));
#8599=CARTESIAN_POINT('',(6.35,-1.9,-3.33));
#8600=CARTESIAN_POINT('',(6.35,-1.9,-3.33));
#8601=CARTESIAN_POINT('',(6.35,-1.9,-3.33));
#8602=CARTESIAN_POINT('Origin',(-6.35,-1.9,-3.33));
#8603=CARTESIAN_POINT('',(-6.35,-1.9,-3.33));
#8604=CARTESIAN_POINT('',(-6.35,-1.9,-3.33));
#8605=CARTESIAN_POINT('',(-6.35,-1.9,-3.33));
#8606=CARTESIAN_POINT('Origin',(-6.35,1.9,-3.33));
#8607=CARTESIAN_POINT('',(-6.35,1.9,-3.33));
#8608=CARTESIAN_POINT('Origin',(0.,0.,-3.33));
#10772=UNCERTAINTY_MEASURE_WITH_UNIT(LENGTH_MEASURE(0.001),#10822,
'DISTANCE_ACCURACY_VALUE',
'Maximum model space distance between geometric entities at asserted c
onnectivities');
#10791=UNCERTAINTY_MEASURE_WITH_UNIT(LENGTH_MEASURE(0.001),#10822,
'DISTANCE_ACCURACY_VALUE',
'Maximum model space distance between geometric entities at asserted c
onnectivities');
#10802=(
GEOMETRIC_REPRESENTATION_CONTEXT(3)
GLOBAL_UNCERTAINTY_ASSIGNED_CONTEXT((#10772))
GLOBAL_UNIT_ASSIGNED_CONTEXT((#10822,#10824,#10825))
REPRESENTATION_CONTEXT('','3D')
);
#10821=(
GEOMETRIC_REPRESENTATION_CONTEXT(3)
GLOBAL_UNCERTAINTY_ASSIGNED_CONTEXT((#10791))
GLOBAL_UNIT_ASSIGNED_CONTEXT((#10822,#10824,#10825))
REPRESENTATION_CONTEXT('','3D')
);
#10822=(
LENGTH_UNIT()
NAMED_UNIT(*)
SI_UNIT(.CENTI.,.METRE.)
);
#10824=(
NAMED_UNIT(*)
PLANE_ANGLE_UNIT()
SI_UNIT($,.RADIAN.)
);
#10825=(
NAMED_UNIT(*)
SI_UNIT($,.STERADIAN.)
SOLID_ANGLE_UNIT()
);
#10836=SHAPE_DEFINITION_REPRESENTATION(#10865,#10934);
#10865=PRODUCT_DEFINITION_SHAPE('',$,#10964);
#10934=SHAPE_REPRESENTATION('',(#5949),#10802);
#10953=PRODUCT_DEFINITION_CONTEXT('part definition',#11042,'design');
#10964=PRODUCT_DEFINITION('Housing','Housing',#10993,#10953);
#10993=PRODUCT_DEFINITION_FORMATION('',$,#11054);
#11042=APPLICATION_CONTEXT(
'Core Data for Automotive Mechanical Design Process');
#11043=PRODUCT_CONTEXT('part definition',#11042,'mechanical');
#11054=PRODUCT('Housing','Housing','Housing',(#11043));
#11108=COLOUR_RGB('Dark Blue',0.08,0.2,0.34);
#11109=FILL_AREA_STYLE_COLOUR('',#11108);
#11110=FILL_AREA_STYLE('',(#11109));
#11111=SURFACE_STYLE_FILL_AREA(#11110);
#11112=SURFACE_SIDE_STYLE('',(#11111));
#11113=SURFACE_STYLE_USAGE(.BOTH.,#11112);
#11114=PRESENTATION_STYLE_ASSIGNMENT((#11113));
ENDSEC;
END-ISO-10303-21;
